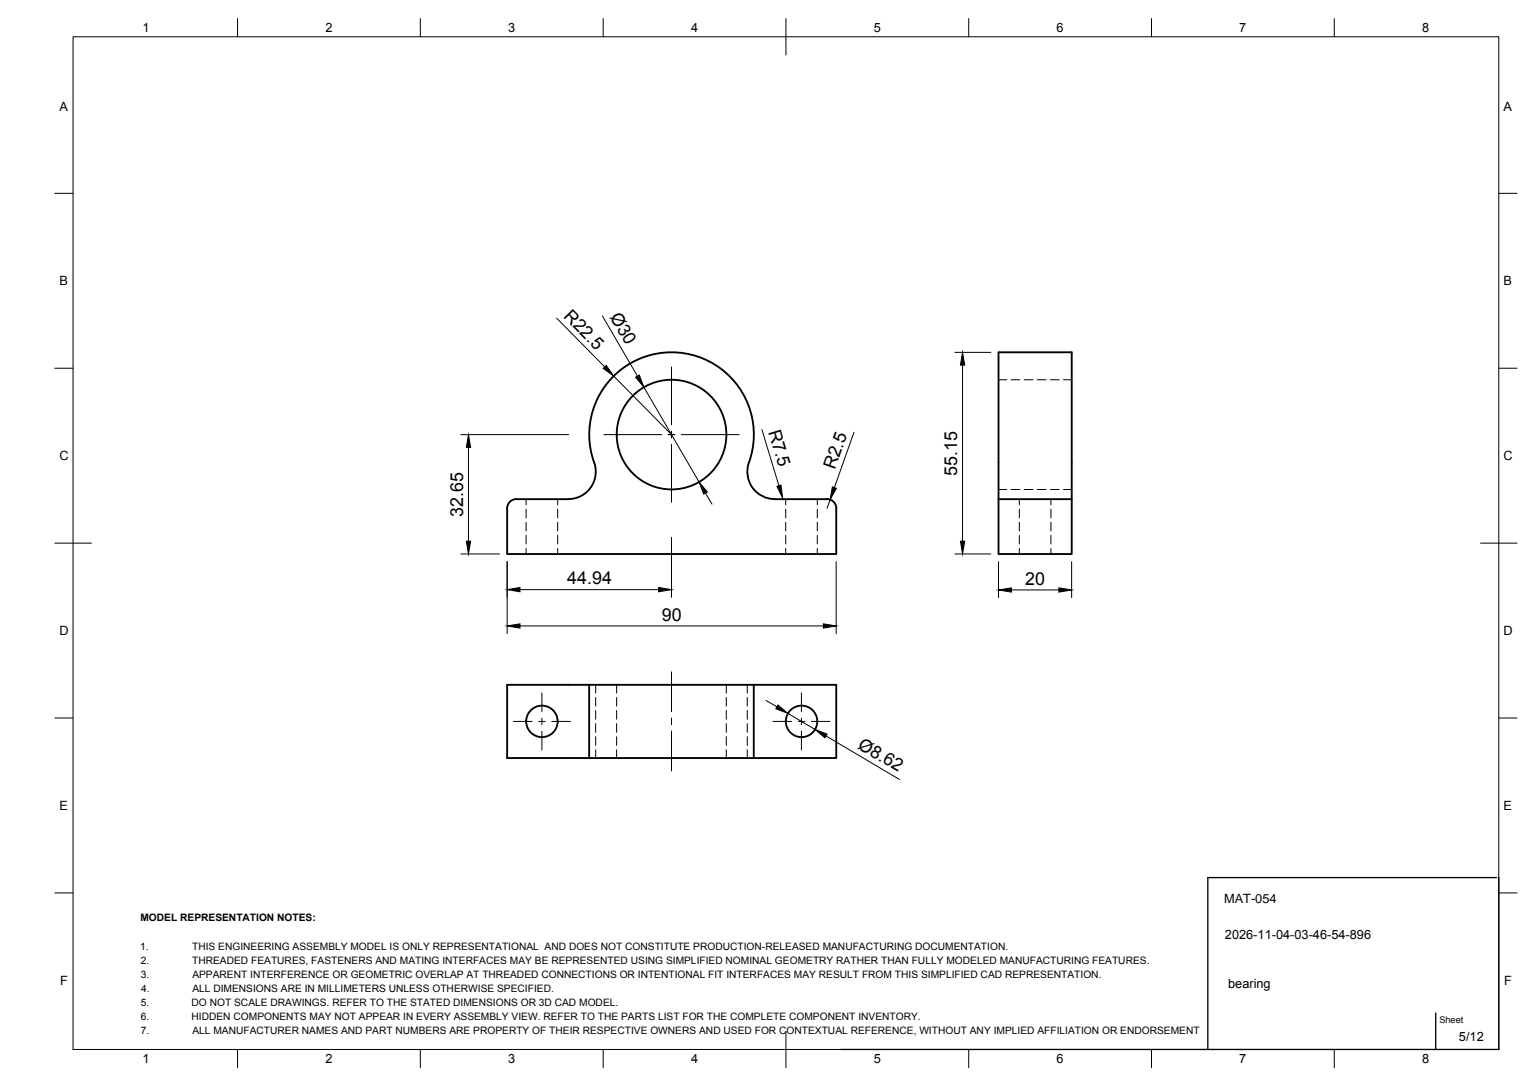
ISO-10303-21;
HEADER;
FILE_DESCRIPTION (('STEP AP214'),
    '1' );
FILE_NAME ('bearing.step',
    '2026-10-21T17:50:41',
    ( '' ),
    ( '' ),
    'SwSTEP 2.0',
    'SolidWorks 2026',
    '' );
FILE_SCHEMA (( 'AUTOMOTIVE_DESIGN' ));
ENDSEC;

DATA;
#98=CYLINDRICAL_SURFACE ( 'NONE', #29121, 7.500000000000000000 ) ;
#144=EDGE_LOOP ( 'NONE', ( #280, #13285, #21736, #21392, #14585, #6579, #11215, #29408, #31879, #667, #8768, #28527, #21247 ) ) ;
#179=DIRECTION ( 'NONE',  ( -0.000000000000000000, -1.000000000000000000, -0.000000000000000000 ) ) ;
#193=DIRECTION ( 'NONE',  ( 0.000000000000000000, -1.000000000000000000, 0.000000000000000000 ) ) ;
#280=ORIENTED_EDGE ( 'NONE', *, *, #30246, .T. ) ;
#297=LINE ( 'NONE', #7943, #15401 ) ;
#335=CARTESIAN_POINT ( 'NONE',  ( 0.000000000000000000, 0.000000000000000000, 0.000000000000000000 ) ) ;
#428=VECTOR ( 'NONE', #33661, 1000.000000000000000 ) ;
#588=ORIENTED_EDGE ( 'NONE', *, *, #13917, .F. ) ;
#650=VECTOR ( 'NONE', #5944, 1000.000000000000000 ) ;
#667=ORIENTED_EDGE ( 'NONE', *, *, #12403, .T. ) ;
#673=AXIS2_PLACEMENT_3D ( 'NONE', #16710, #32352, #5290 ) ;
#720=CIRCLE ( 'NONE', #7507, 7.500000000000000000 ) ;
#754=DIRECTION ( 'NONE',  ( 0.000000000000000000, 0.000000000000000000, 1.000000000000000000 ) ) ;
#776=DIRECTION ( 'NONE',  ( 0.000000000000000000, -1.000000000000000000, 0.000000000000000000 ) ) ;
#987=AXIS2_PLACEMENT_3D ( 'NONE', #7647, #179, #11034 ) ;
#1067=LINE ( 'NONE', #27933, #15226 ) ;
#1089=ORIENTED_EDGE ( 'NONE', *, *, #19291, .F. ) ;
#1148=DIRECTION ( 'NONE',  ( 1.000000000000000000, 0.000000000000000000, 0.000000000000000000 ) ) ;
#1179=FACE_BOUND ( 'NONE', #11958, .T. ) ;
#1196=DIRECTION ( 'NONE',  ( 0.000000000000000000, -1.000000000000000000, 0.000000000000000000 ) ) ;
#1238=CARTESIAN_POINT ( 'NONE',  ( 20.73027531293552528, -10.15143121711728469, 0.000000000000000000 ) ) ;
#1246=VERTEX_POINT ( 'NONE', #33189 ) ;
#1310=DIRECTION ( 'NONE',  ( 1.000000000000000000, 0.000000000000000000, -0.000000000000000000 ) ) ;
#1315=VERTEX_POINT ( 'NONE', #22523 ) ;
#1337=VERTEX_POINT ( 'NONE', #20892 ) ;
#1417=CARTESIAN_POINT ( 'NONE',  ( -35.55956070192387841, -32.65143121711728469, 14.30932821646982411 ) ) ;
#1464=ORIENTED_EDGE ( 'NONE', *, *, #2512, .T. ) ;
#1554=CIRCLE ( 'NONE', #28261, 4.309328216469825001 ) ;
#1579=DIRECTION ( 'NONE',  ( 0.000000000000000000, 0.000000000000000000, 1.000000000000000000 ) ) ;
#1590=CARTESIAN_POINT ( 'NONE',  ( 42.44043929807611448, -17.65143121711728469, 0.000000000000000000 ) ) ;
#1602=CARTESIAN_POINT ( 'NONE',  ( -45.05956070192387841, -32.65143121711728469, 20.00000000000000000 ) ) ;
#1647=EDGE_LOOP ( 'NONE', ( #35054, #12511, #7318, #1089 ) ) ;
#1650=FACE_OUTER_BOUND ( 'NONE', #15361, .T. ) ;
#1682=ORIENTED_EDGE ( 'NONE', *, *, #28659, .T. ) ;
#1703=LINE ( 'NONE', #15247, #2230 ) ;
#1786=ORIENTED_EDGE ( 'NONE', *, *, #28659, .F. ) ;
#1868=CARTESIAN_POINT ( 'NONE',  ( -42.55956070192386420, -17.65143121711728469, 0.000000000000000000 ) ) ;
#1884=FACE_OUTER_BOUND ( 'NONE', #34354, .T. ) ;
#1887=FACE_BOUND ( 'NONE', #19466, .T. ) ;
#1934=EDGE_LOOP ( 'NONE', ( #11019, #16399, #2768, #7931 ) ) ;
#1951=LINE ( 'NONE', #13005, #5578 ) ;
#2024=CIRCLE ( 'NONE', #9434, 7.500000000000000000 ) ;
#2056=VECTOR ( 'NONE', #12798, 1000.000000000000000 ) ;
#2062=ORIENTED_EDGE ( 'NONE', *, *, #16987, .T. ) ;
#2158=ADVANCED_FACE ( 'NONE', ( #26680 ), #13166, .F. ) ;
#2194=DIRECTION ( 'NONE',  ( -1.000000000000000000, 0.000000000000000000, 0.000000000000000000 ) ) ;
#2200=DIRECTION ( 'NONE',  ( 0.000000000000000000, 0.000000000000000000, 1.000000000000000000 ) ) ;
#2230=VECTOR ( 'NONE', #34272, 1000.000000000000000 ) ;
#2289=ORIENTED_EDGE ( 'NONE', *, *, #33790, .T. ) ;
#2360=AXIS2_PLACEMENT_3D ( 'NONE', #13291, #2588, #10616 ) ;
#2374=ORIENTED_EDGE ( 'NONE', *, *, #13917, .T. ) ;
#2424=ORIENTED_EDGE ( 'NONE', *, *, #14612, .T. ) ;
#2505=CIRCLE ( 'NONE', #31479, 15.00000000000000000 ) ;
#2512=EDGE_CURVE ( 'NONE', #15960, #1246, #1554, .T. ) ;
#2588=DIRECTION ( 'NONE',  ( -0.000000000000000000, -0.000000000000000000, -1.000000000000000000 ) ) ;
#2665=FACE_OUTER_BOUND ( 'NONE', #32945, .T. ) ;
#2768=ORIENTED_EDGE ( 'NONE', *, *, #19291, .T. ) ;
#2784=CARTESIAN_POINT ( 'NONE',  ( 42.44043929807611448, -20.15143121711728469, 20.00000000000000000 ) ) ;
#2906=FACE_OUTER_BOUND ( 'NONE', #15377, .T. ) ;
#3005=ORIENTED_EDGE ( 'NONE', *, *, #26043, .F. ) ;
#3145=DIRECTION ( 'NONE',  ( -0.000000000000000000, -0.000000000000000000, -1.000000000000000000 ) ) ;
#3170=DIRECTION ( 'NONE',  ( 0.000000000000000000, 0.000000000000000000, -1.000000000000000000 ) ) ;
#3183=ORIENTED_EDGE ( 'NONE', *, *, #29865, .T. ) ;
#3190=VECTOR ( 'NONE', #5924, 1000.000000000000000 ) ;
#3214=SHAPE_DEFINITION_REPRESENTATION ( #3232, #11185 ) ;
#3232=PRODUCT_DEFINITION_SHAPE ( 'NONE', 'NONE',  #30332 ) ;
#3267=DIRECTION ( 'NONE',  ( -0.000000000000000000, -0.000000000000000000, -1.000000000000000000 ) ) ;
#3274=LINE ( 'NONE', #11658, #4499 ) ;
#3536=DIRECTION ( 'NONE',  ( 1.000000000000000000, 0.000000000000000000, 0.000000000000000000 ) ) ;
#3537=ORIENTED_EDGE ( 'NONE', *, *, #17476, .T. ) ;
#3726=EDGE_CURVE ( 'NONE', #14044, #25632, #1951, .T. ) ;
#3731=VECTOR ( 'NONE', #32637, 1000.000000000000000 ) ;
#3774=CIRCLE ( 'NONE', #26508, 4.309328216469825001 ) ;
#3834=CIRCLE ( 'NONE', #33395, 4.309328216469825001 ) ;
#4017=FACE_BOUND ( 'NONE', #34001, .T. ) ;
#4073=CIRCLE ( 'NONE', #6902, 7.500000000000000000 ) ;
#4099=CARTESIAN_POINT ( 'NONE',  ( -42.55956070192386420, -17.65143121711728469, 20.00000000000000000 ) ) ;
#4161=CARTESIAN_POINT ( 'NONE',  ( 0.000000000000000000, 0.000000000000000000, 20.00000000000000000 ) ) ;
#4275=CARTESIAN_POINT ( 'NONE',  ( 0.000000000000000000, 0.000000000000000000, 20.00000000000000000 ) ) ;
#4282=DIRECTION ( 'NONE',  ( 0.000000000000000000, 0.000000000000000000, 1.000000000000000000 ) ) ;
#4476=CYLINDRICAL_SURFACE ( 'NONE', #23230, 7.500000000000000000 ) ;
#4482=DIRECTION ( 'NONE',  ( 0.000000000000000000, 1.000000000000000000, 0.000000000000000000 ) ) ;
#4499=VECTOR ( 'NONE', #5934, 1000.000000000000000 ) ;
#4571=VERTEX_POINT ( 'NONE', #32067 ) ;
#4572=CARTESIAN_POINT ( 'NONE',  ( -42.55956070192386420, -17.65143121711728469, 0.000000000000000000 ) ) ;
#4576=FACE_OUTER_BOUND ( 'NONE', #1934, .T. ) ;
#4606=VERTEX_POINT ( 'NONE', #26730 ) ;
#4611=DIRECTION ( 'NONE',  ( 0.000000000000000000, 0.000000000000000000, 1.000000000000000000 ) ) ;
#4856=CARTESIAN_POINT ( 'NONE',  ( -28.23027531293552528, -10.15143121711728469, 20.00000000000000000 ) ) ;
#4884=AXIS2_PLACEMENT_3D ( 'NONE', #10644, #13141, #23974 ) ;
#4893=EDGE_LOOP ( 'NONE', ( #17206, #26632 ) ) ;
#4899=DIRECTION ( 'NONE',  ( -0.000000000000000000, -0.000000000000000000, -1.000000000000000000 ) ) ;
#4963=ORIENTED_EDGE ( 'NONE', *, *, #20775, .T. ) ;
#5064=CARTESIAN_POINT ( 'NONE',  ( 44.94043929807611448, -32.65143121711728469, 20.00000000000000000 ) ) ;
#5074=CYLINDRICAL_SURFACE ( 'NONE', #6927, 4.309328216469825001 ) ;
#5186=DIRECTION ( 'NONE',  ( -0.000000000000000000, -1.000000000000000000, -0.000000000000000000 ) ) ;
#5189=EDGE_CURVE ( 'NONE', #20760, #34690, #26627, .T. ) ;
#5290=DIRECTION ( 'NONE',  ( 1.000000000000000000, 0.000000000000000000, 0.000000000000000000 ) ) ;
#5355=EDGE_LOOP ( 'NONE', ( #4963, #33386, #10408, #3537 ) ) ;
#5426=DIRECTION ( 'NONE',  ( -1.000000000000000000, 0.000000000000000000, 0.000000000000000000 ) ) ;
#5445=ORIENTED_EDGE ( 'NONE', *, *, #19569, .F. ) ;
#5578=VECTOR ( 'NONE', #23841, 1000.000000000000000 ) ;
#5591=CYLINDRICAL_SURFACE ( 'NONE', #25040, 4.309328216469825001 ) ;
#5624=EDGE_CURVE ( 'NONE', #17462, #1337, #3834, .T. ) ;
#5658=LINE ( 'NONE', #32062, #17725 ) ;
#5665=DIRECTION ( 'NONE',  ( 1.000000000000000000, 0.000000000000000000, 0.000000000000000000 ) ) ;
#5735=CIRCLE ( 'NONE', #12609, 7.500000000000000000 ) ;
#5746=AXIS2_PLACEMENT_3D ( 'NONE', #13699, #29902, #5665 ) ;
#5924=DIRECTION ( 'NONE',  ( -0.000000000000000000, -0.000000000000000000, -1.000000000000000000 ) ) ;
#5934=DIRECTION ( 'NONE',  ( 1.000000000000000000, 0.000000000000000000, 0.000000000000000000 ) ) ;
#5944=DIRECTION ( 'NONE',  ( -0.000000000000000000, -0.000000000000000000, -1.000000000000000000 ) ) ;
#5953=VECTOR ( 'NONE', #24547, 1000.000000000000000 ) ;
#5995=ORIENTED_EDGE ( 'NONE', *, *, #7093, .F. ) ;
#6095=VECTOR ( 'NONE', #4482, 1000.000000000000000 ) ;
#6135=ORIENTED_EDGE ( 'NONE', *, *, #30246, .F. ) ;
#6166=EDGE_CURVE ( 'NONE', #30767, #27908, #24708, .T. ) ;
#6275=DIRECTION ( 'NONE',  ( -1.000000000000000000, 0.000000000000000000, 0.000000000000000000 ) ) ;
#6422=ORIENTED_EDGE ( 'NONE', *, *, #5189, .T. ) ;
#6476=DIRECTION ( 'NONE',  ( 0.000000000000000000, 0.000000000000000000, -1.000000000000000000 ) ) ;
#6579=ORIENTED_EDGE ( 'NONE', *, *, #35041, .T. ) ;
#6732=AXIS2_PLACEMENT_3D ( 'NONE', #11381, #11213, #30241 ) ;
#6779=LINE ( 'NONE', #31683, #25200 ) ;
#6823=DIRECTION ( 'NONE',  ( 0.000000000000000000, 0.000000000000000000, 1.000000000000000000 ) ) ;
#6879=AXIS2_PLACEMENT_3D ( 'NONE', #14649, #22815, #9288 ) ;
#6902=AXIS2_PLACEMENT_3D ( 'NONE', #14201, #3145, #22373 ) ;
#6904=ADVANCED_FACE ( 'NONE', ( #17929, #1179, #20062 ), #28755, .F. ) ;
#6907=ORIENTED_EDGE ( 'NONE', *, *, #26043, .T. ) ;
#6926=CARTESIAN_POINT ( 'NONE',  ( 44.94043929807611448, -20.15143121711728469, 20.00000000000000000 ) ) ;
#6927=AXIS2_PLACEMENT_3D ( 'NONE', #15795, #26623, #10431 ) ;
#6956=PLANE ( 'NONE',  #7053 ) ;
#7022=DIRECTION ( 'NONE',  ( 0.000000000000000000, -1.000000000000000000, 0.000000000000000000 ) ) ;
#7048=ORIENTED_EDGE ( 'NONE', *, *, #7445, .F. ) ;
#7053=AXIS2_PLACEMENT_3D ( 'NONE', #17847, #28681, #4282 ) ;
#7057=ORIENTED_EDGE ( 'NONE', *, *, #10691, .T. ) ;
#7075=LINE ( 'NONE', #9239, #10341 ) ;
#7093=EDGE_CURVE ( 'NONE', #11385, #31447, #18617, .T. ) ;
#7134=ORIENTED_EDGE ( 'NONE', *, *, #31070, .T. ) ;
#7156=CYLINDRICAL_SURFACE ( 'NONE', #27609, 2.500000000000002220 ) ;
#7177=DIRECTION ( 'NONE',  ( -1.000000000000000000, 0.000000000000000000, 0.000000000000000000 ) ) ;
#7238=EDGE_CURVE ( 'NONE', #29888, #25980, #21788, .T. ) ;
#7318=ORIENTED_EDGE ( 'NONE', *, *, #16987, .F. ) ;
#7422=CARTESIAN_POINT ( 'NONE',  ( -35.55956070192387841, -32.65143121711728469, 5.690671783530174999 ) ) ;
#7443=ADVANCED_FACE ( 'NONE', ( #29590 ), #7156, .T. ) ;
#7444=CARTESIAN_POINT ( 'NONE',  ( 20.73027531293552528, -10.15143121711728469, 20.00000000000000000 ) ) ;
#7445=EDGE_CURVE ( 'NONE', #1337, #23936, #18061, .T. ) ;
#7470=CARTESIAN_POINT ( 'NONE',  ( 28.23027531293552528, -17.65143121711728469, 20.00000000000000000 ) ) ;
#7507=AXIS2_PLACEMENT_3D ( 'NONE', #4856, #33412, #17247 ) ;
#7509=DIRECTION ( 'NONE',  ( -0.000000000000000000, -0.000000000000000000, -1.000000000000000000 ) ) ;
#7524=VERTEX_POINT ( 'NONE', #31724 ) ;
#7588=CARTESIAN_POINT ( 'NONE',  ( -28.23027531293552528, -17.65143121711728469, 0.000000000000000000 ) ) ;
#7601=ORIENTED_EDGE ( 'NONE', *, *, #32770, .T. ) ;
#7647=CARTESIAN_POINT ( 'NONE',  ( -35.55956070192387841, -12.65143121711728291, 10.00000000000000000 ) ) ;
#7706=FACE_OUTER_BOUND ( 'NONE', #21398, .T. ) ;
#7751=FACE_OUTER_BOUND ( 'NONE', #24508, .T. ) ;
#7754=EDGE_CURVE ( 'NONE', #25273, #4606, #23458, .T. ) ;
#7759=VERTEX_POINT ( 'NONE', #7422 ) ;
#7760=CARTESIAN_POINT ( 'NONE',  ( 44.94043929807611448, -32.65143121711728469, 20.00000000000000000 ) ) ;
#7854=EDGE_CURVE ( 'NONE', #1246, #15960, #21952, .T. ) ;
#7931=ORIENTED_EDGE ( 'NONE', *, *, #32770, .F. ) ;
#7943=CARTESIAN_POINT ( 'NONE',  ( -28.23027531293552528, -17.65143121711728469, 20.00000000000000000 ) ) ;
#7968=DIRECTION ( 'NONE',  ( -0.000000000000000000, -0.000000000000000000, -1.000000000000000000 ) ) ;
#8026=CIRCLE ( 'NONE', #22831, 22.50000000000000355 ) ;
#8101=EDGE_CURVE ( 'NONE', #23708, #12488, #31623, .T. ) ;
#8204=( LENGTH_UNIT ( ) NAMED_UNIT ( * ) SI_UNIT ( .MILLI., .METRE. ) );
#8240=ORIENTED_EDGE ( 'NONE', *, *, #27319, .F. ) ;
#8255=FACE_OUTER_BOUND ( 'NONE', #9278, .T. ) ;
#8459=CIRCLE ( 'NONE', #32889, 15.00000000000000000 ) ;
#8477=ORIENTED_EDGE ( 'NONE', *, *, #9298, .F. ) ;
#8589=ORIENTED_EDGE ( 'NONE', *, *, #15548, .F. ) ;
#8658=DIRECTION ( 'NONE',  ( 0.000000000000000000, 0.000000000000000000, 1.000000000000000000 ) ) ;
#8665=AXIS2_PLACEMENT_3D ( 'NONE', #21239, #27510, #2194 ) ;
#8673=CARTESIAN_POINT ( 'NONE',  ( -45.05956070192387841, -20.15143121711730245, 0.000000000000000000 ) ) ;
#8704=EDGE_CURVE ( 'NONE', #27908, #4571, #12193, .T. ) ;
#8709=DIRECTION ( 'NONE',  ( 0.000000000000000000, 0.000000000000000000, -1.000000000000000000 ) ) ;
#8768=ORIENTED_EDGE ( 'NONE', *, *, #7754, .T. ) ;
#8858=VECTOR ( 'NONE', #28004, 1000.000000000000000 ) ;
#9037=STYLED_ITEM('',(#35275),#10712);
#9038=EDGE_CURVE ( 'NONE', #26426, #14044, #15163, .T. ) ;
#9046=DIRECTION ( 'NONE',  ( -0.000000000000000000, -1.000000000000000000, -0.000000000000000000 ) ) ;
#9063=DIRECTION ( 'NONE',  ( -1.000000000000000000, -0.000000000000000000, -0.000000000000000000 ) ) ;
#9153=AXIS2_PLACEMENT_3D ( 'NONE', #12764, #9563, #18280 ) ;
#9239=CARTESIAN_POINT ( 'NONE',  ( -42.55956070192386420, -17.65143121711728469, 20.00000000000000000 ) ) ;
#9278=EDGE_LOOP ( 'NONE', ( #3183, #24989, #30938, #30551 ) ) ;
#9288=DIRECTION ( 'NONE',  ( -1.000000000000000000, 0.000000000000000000, 0.000000000000000000 ) ) ;
#9298=EDGE_CURVE ( 'NONE', #25980, #7524, #24542, .T. ) ;
#9371=AXIS2_PLACEMENT_3D ( 'NONE', #23997, #9046, #3170 ) ;
#9421=CARTESIAN_POINT ( 'NONE',  ( -45.05956070192387841, -32.65143121711728469, 20.00000000000000000 ) ) ;
#9434=AXIS2_PLACEMENT_3D ( 'NONE', #10634, #15983, #18825 ) ;
#9505=CARTESIAN_POINT ( 'NONE',  ( 44.94043929807611448, -20.15143121711728469, 0.000000000000000000 ) ) ;
#9535=EDGE_CURVE ( 'NONE', #33194, #31447, #1067, .T. ) ;
#9563=DIRECTION ( 'NONE',  ( -0.000000000000000000, 0.000000000000000000, -1.000000000000000000 ) ) ;
#9610=CARTESIAN_POINT ( 'NONE',  ( -45.05956070192387841, -20.15143121711730245, 0.000000000000000000 ) ) ;
#9779=ORIENTED_EDGE ( 'NONE', *, *, #29342, .T. ) ;
#9841=LINE ( 'NONE', #23542, #6095 ) ;
#9842=CARTESIAN_POINT ( 'NONE',  ( -42.55956070192387841, -20.15143121711728469, 20.00000000000000000 ) ) ;
#9855=CYLINDRICAL_SURFACE ( 'NONE', #8665, 22.50000000000000355 ) ;
#9862=DIRECTION ( 'NONE',  ( 0.000000000000000000, -1.000000000000000000, 0.000000000000000000 ) ) ;
#9884=PRODUCT_DEFINITION_FORMATION_WITH_SPECIFIED_SOURCE ( 'ANY', '', #16613, .NOT_KNOWN. ) ;
#9992=VERTEX_POINT ( 'NONE', #7444 ) ;
#10012=CARTESIAN_POINT ( 'NONE',  ( -35.55956070192387841, -32.65143121711728469, 10.00000000000000000 ) ) ;
#10085=ORIENTED_EDGE ( 'NONE', *, *, #5624, .F. ) ;
#10100=FACE_OUTER_BOUND ( 'NONE', #1647, .T. ) ;
#10195=CARTESIAN_POINT ( 'NONE',  ( 42.44043929807611448, -17.65143121711728469, 20.00000000000000000 ) ) ;
#10202=CARTESIAN_POINT ( 'NONE',  ( -45.05956070192387841, -32.65143121711728469, 0.000000000000000000 ) ) ;
#10261=ORIENTED_EDGE ( 'NONE', *, *, #24371, .F. ) ;
#10271=DIRECTION ( 'NONE',  ( -1.000000000000000000, 0.000000000000000000, 0.000000000000000000 ) ) ;
#10293=CARTESIAN_POINT ( 'NONE',  ( 0.000000000000000000, 0.000000000000000000, 20.00000000000000000 ) ) ;
#10341=VECTOR ( 'NONE', #9063, 1000.000000000000000 ) ;
#10358=EDGE_LOOP ( 'NONE', ( #28928, #26404, #12720, #20054 ) ) ;
#10408=ORIENTED_EDGE ( 'NONE', *, *, #7754, .F. ) ;
#10431=DIRECTION ( 'NONE',  ( 0.000000000000000000, 0.000000000000000000, -1.000000000000000000 ) ) ;
#10543=( NAMED_UNIT ( * ) PLANE_ANGLE_UNIT ( ) SI_UNIT ( $, .RADIAN. ) );
#10581=EDGE_LOOP ( 'NONE', ( #8589, #12296, #11638, #8240 ) ) ;
#10616=DIRECTION ( 'NONE',  ( -1.000000000000000000, 0.000000000000000000, 0.000000000000000000 ) ) ;
#10634=CARTESIAN_POINT ( 'NONE',  ( 28.23027531293552528, -10.15143121711728469, 0.000000000000000000 ) ) ;
#10644=CARTESIAN_POINT ( 'NONE',  ( 35.44043929807611448, -17.65143121711728469, 10.00000000000000000 ) ) ;
#10669=DIRECTION ( 'NONE',  ( 0.000000000000000000, 0.000000000000000000, 1.000000000000000000 ) ) ;
#10677=ORIENTED_EDGE ( 'NONE', *, *, #9535, .F. ) ;
#10691=EDGE_CURVE ( 'NONE', #16381, #1315, #15322, .T. ) ;
#10712=MANIFOLD_SOLID_BREP ( 'Cut-Extrude1', #29869 ) ;
#10929=( GEOMETRIC_REPRESENTATION_CONTEXT ( 3 ) GLOBAL_UNCERTAINTY_ASSIGNED_CONTEXT ( ( #28468 ) ) GLOBAL_UNIT_ASSIGNED_CONTEXT ( ( #14663, #30490, #31015 ) ) REPRESENTATION_CONTEXT ( 'NONE', 'WORKASPACE' ) );
#11019=ORIENTED_EDGE ( 'NONE', *, *, #8704, .F. ) ;
#11034=DIRECTION ( 'NONE',  ( 0.000000000000000000, 0.000000000000000000, -1.000000000000000000 ) ) ;
#11068=( NAMED_UNIT ( * ) SI_UNIT ( $, .STERADIAN. ) SOLID_ANGLE_UNIT ( ) );
#11140=LINE ( 'NONE', #33538, #650 ) ;
#11171=ORIENTED_EDGE ( 'NONE', *, *, #7093, .T. ) ;
#11185=SHAPE_REPRESENTATION ( 'bearing', ( #28566 ), #10929 ) ;
#11213=DIRECTION ( 'NONE',  ( 0.000000000000000000, 0.000000000000000000, 1.000000000000000000 ) ) ;
#11215=ORIENTED_EDGE ( 'NONE', *, *, #30006, .T. ) ;
#11232=DIRECTION ( 'NONE',  ( 0.000000000000000000, 0.000000000000000000, -1.000000000000000000 ) ) ;
#11298=CARTESIAN_POINT ( 'NONE',  ( 28.23027531293552528, -17.65143121711728469, 20.00000000000000000 ) ) ;
#11330=ADVANCED_FACE ( 'NONE', ( #10100 ), #18307, .F. ) ;
#11332=( GEOMETRIC_REPRESENTATION_CONTEXT ( 3 ) GLOBAL_UNCERTAINTY_ASSIGNED_CONTEXT ( ( #31933 ) ) GLOBAL_UNIT_ASSIGNED_CONTEXT ( ( #8204, #10543, #11068 ) ) REPRESENTATION_CONTEXT ( 'NONE', 'WORKASPACE' ) );
#11381=CARTESIAN_POINT ( 'NONE',  ( 42.44043929807611448, -20.15143121711728469, 0.000000000000000000 ) ) ;
#11385=VERTEX_POINT ( 'NONE', #7588 ) ;
#11495=AXIS2_PLACEMENT_3D ( 'NONE', #30693, #24981, #1148 ) ;
#11619=FACE_OUTER_BOUND ( 'NONE', #144, .T. ) ;
#11636=EDGE_LOOP ( 'NONE', ( #29071, #13902, #19431, #7057 ) ) ;
#11638=ORIENTED_EDGE ( 'NONE', *, *, #18730, .T. ) ;
#11658=CARTESIAN_POINT ( 'NONE',  ( -45.05956070192387841, -32.65143121711728469, 0.000000000000000000 ) ) ;
#11690=ORIENTED_EDGE ( 'NONE', *, *, #15800, .F. ) ;
#11754=DIRECTION ( 'NONE',  ( 0.000000000000000000, -1.000000000000000000, 0.000000000000000000 ) ) ;
#11833=LINE ( 'NONE', #16643, #8858 ) ;
#11844=CARTESIAN_POINT ( 'NONE',  ( 15.00000000000000000, 1.836970198721029589E-15, 20.00000000000000000 ) ) ;
#11955=VECTOR ( 'NONE', #32052, 1000.000000000000000 ) ;
#11958=EDGE_LOOP ( 'NONE', ( #1786, #32913 ) ) ;
#11980=ADVANCED_FACE ( 'NONE', ( #2906 ), #27653, .T. ) ;
#12006=CIRCLE ( 'NONE', #17143, 4.309328216469825001 ) ;
#12034=ADVANCED_FACE ( 'NONE', ( #25862 ), #33695, .F. ) ;
#12058=ADVANCED_FACE ( 'NONE', ( #1650 ), #4476, .F. ) ;
#12193=LINE ( 'NONE', #11844, #13398 ) ;
#12248=PLANE ( 'NONE',  #9153 ) ;
#12252=CARTESIAN_POINT ( 'NONE',  ( -42.55956070192386420, -17.65143121711728469, 20.00000000000000000 ) ) ;
#12296=ORIENTED_EDGE ( 'NONE', *, *, #13818, .T. ) ;
#12403=EDGE_CURVE ( 'NONE', #14044, #25273, #30948, .T. ) ;
#12449=CARTESIAN_POINT ( 'NONE',  ( -21.17270648470164218, -7.613573412837966181, 20.00000000000000000 ) ) ;
#12488=VERTEX_POINT ( 'NONE', #12449 ) ;
#12491=DIRECTION ( 'NONE',  ( 1.000000000000000000, 0.000000000000000000, 0.000000000000000000 ) ) ;
#12511=ORIENTED_EDGE ( 'NONE', *, *, #8704, .T. ) ;
#12519=CARTESIAN_POINT ( 'NONE',  ( 28.23027531293552528, -10.15143121711728469, 20.00000000000000000 ) ) ;
#12564=DIRECTION ( 'NONE',  ( 0.000000000000000000, 0.000000000000000000, 1.000000000000000000 ) ) ;
#12609=AXIS2_PLACEMENT_3D ( 'NONE', #34128, #20273, #17448 ) ;
#12720=ORIENTED_EDGE ( 'NONE', *, *, #30005, .F. ) ;
#12764=CARTESIAN_POINT ( 'NONE',  ( 28.23027531293552528, -10.15143121711728469, 0.000000000000000000 ) ) ;
#12768=FACE_OUTER_BOUND ( 'NONE', #15181, .T. ) ;
#12798=DIRECTION ( 'NONE',  ( 0.000000000000000000, 1.000000000000000000, 0.000000000000000000 ) ) ;
#12799=EDGE_CURVE ( 'NONE', #27908, #30767, #8459, .T. ) ;
#12846=DIRECTION ( 'NONE',  ( -0.000000000000000000, -1.000000000000000000, -0.000000000000000000 ) ) ;
#12907=EDGE_CURVE ( 'NONE', #12488, #32903, #1703, .T. ) ;
#13005=CARTESIAN_POINT ( 'NONE',  ( -45.05956070192387841, -32.65143121711728469, 20.00000000000000000 ) ) ;
#13052=DIRECTION ( 'NONE',  ( -0.000000000000000000, -0.000000000000000000, -1.000000000000000000 ) ) ;
#13073=DIRECTION ( 'NONE',  ( 1.000000000000000000, 0.000000000000000000, 0.000000000000000000 ) ) ;
#13093=VECTOR ( 'NONE', #21913, 1000.000000000000000 ) ;
#13141=DIRECTION ( 'NONE',  ( 0.000000000000000000, -1.000000000000000000, 0.000000000000000000 ) ) ;
#13144=EDGE_CURVE ( 'NONE', #25632, #15499, #3274, .T. ) ;
#13166=CYLINDRICAL_SURFACE ( 'NONE', #9371, 4.309328216469825001 ) ;
#13205=FACE_OUTER_BOUND ( 'NONE', #11636, .T. ) ;
#13212=CARTESIAN_POINT ( 'NONE',  ( 20.73027531293552528, -10.15143121711728469, 20.00000000000000000 ) ) ;
#13219=DIRECTION ( 'NONE',  ( 0.000000000000000000, 0.000000000000000000, -1.000000000000000000 ) ) ;
#13250=AXIS2_PLACEMENT_3D ( 'NONE', #22071, #11754, #8709 ) ;
#13285=ORIENTED_EDGE ( 'NONE', *, *, #15548, .T. ) ;
#13291=CARTESIAN_POINT ( 'NONE',  ( 42.44043929807611448, -20.15143121711728469, 20.00000000000000000 ) ) ;
#13398=VECTOR ( 'NONE', #33529, 1000.000000000000000 ) ;
#13457=FACE_OUTER_BOUND ( 'NONE', #28066, .T. ) ;
#13479=DIRECTION ( 'NONE',  ( -1.000000000000000000, 0.000000000000000000, 0.000000000000000000 ) ) ;
#13697=ORIENTED_EDGE ( 'NONE', *, *, #8101, .F. ) ;
#13699=CARTESIAN_POINT ( 'NONE',  ( -28.23027531293552528, -10.15143121711728469, 0.000000000000000000 ) ) ;
#13700=VERTEX_POINT ( 'NONE', #14834 ) ;
#13818=EDGE_CURVE ( 'NONE', #9992, #23016, #29221, .T. ) ;
#13851=ORIENTED_EDGE ( 'NONE', *, *, #5189, .F. ) ;
#13902=ORIENTED_EDGE ( 'NONE', *, *, #22751, .F. ) ;
#13917=EDGE_CURVE ( 'NONE', #17462, #7759, #27774, .T. ) ;
#14026=EDGE_CURVE ( 'NONE', #4606, #20760, #22968, .T. ) ;
#14036=DIRECTION ( 'NONE',  ( 1.000000000000000000, 0.000000000000000000, 0.000000000000000000 ) ) ;
#14044=VERTEX_POINT ( 'NONE', #1602 ) ;
#14102=VERTEX_POINT ( 'NONE', #28313 ) ;
#14201=CARTESIAN_POINT ( 'NONE',  ( 28.23027531293552528, -10.15143121711728469, 20.00000000000000000 ) ) ;
#14349=AXIS2_PLACEMENT_3D ( 'NONE', #2784, #18828, #13479 ) ;
#14500=DIRECTION ( 'NONE',  ( -1.000000000000000000, 0.000000000000000000, 0.000000000000000000 ) ) ;
#14585=ORIENTED_EDGE ( 'NONE', *, *, #8101, .T. ) ;
#14612=EDGE_CURVE ( 'NONE', #18684, #11385, #297, .T. ) ;
#14649=CARTESIAN_POINT ( 'NONE',  ( 28.23027531293552528, -10.15143121711728469, 20.00000000000000000 ) ) ;
#14663=( LENGTH_UNIT ( ) NAMED_UNIT ( * ) SI_UNIT ( .MILLI., .METRE. ) );
#14730=DIRECTION ( 'NONE',  ( 0.000000000000000000, 1.000000000000000000, 0.000000000000000000 ) ) ;
#14833=VECTOR ( 'NONE', #15910, 1000.000000000000000 ) ;
#14834=CARTESIAN_POINT ( 'NONE',  ( 22.50000000000000355, 2.755455298081545172E-15, 20.00000000000000000 ) ) ;
#14862=CARTESIAN_POINT ( 'NONE',  ( -15.00000000000000000, 0.000000000000000000, 20.00000000000000000 ) ) ;
#14946=EDGE_LOOP ( 'NONE', ( #34225, #32974, #6907, #1682 ) ) ;
#15050=DIRECTION ( 'NONE',  ( -0.000000000000000000, -0.000000000000000000, -1.000000000000000000 ) ) ;
#15068=CARTESIAN_POINT ( 'NONE',  ( -35.55956070192387841, -17.65143121711728469, 10.00000000000000000 ) ) ;
#15080=EDGE_CURVE ( 'NONE', #1337, #17462, #12006, .T. ) ;
#15127=CARTESIAN_POINT ( 'NONE',  ( -45.05956070192387841, -20.15143121711730245, 20.00000000000000000 ) ) ;
#15163=LINE ( 'NONE', #27972, #428 ) ;
#15181=EDGE_LOOP ( 'NONE', ( #11171, #10677, #27068, #2424 ) ) ;
#15226=VECTOR ( 'NONE', #22776, 1000.000000000000000 ) ;
#15244=ORIENTED_EDGE ( 'NONE', *, *, #29080, .F. ) ;
#15245=CARTESIAN_POINT ( 'NONE',  ( -45.05956070192387841, -32.65143121711728469, 20.00000000000000000 ) ) ;
#15247=CARTESIAN_POINT ( 'NONE',  ( -21.17270648470164218, -7.613573412837966181, 20.00000000000000000 ) ) ;
#15258=ORIENTED_EDGE ( 'NONE', *, *, #7445, .T. ) ;
#15272=ORIENTED_EDGE ( 'NONE', *, *, #13144, .F. ) ;
#15322=CIRCLE ( 'NONE', #27223, 22.50000000000000355 ) ;
#15361=EDGE_LOOP ( 'NONE', ( #31637, #6135, #15564, #24418 ) ) ;
#15377=EDGE_LOOP ( 'NONE', ( #22640, #17518, #27219, #21030 ) ) ;
#15401=VECTOR ( 'NONE', #24473, 1000.000000000000000 ) ;
#15404=EDGE_CURVE ( 'NONE', #34690, #7524, #5658, .T. ) ;
#15499=VERTEX_POINT ( 'NONE', #28276 ) ;
#15548=EDGE_CURVE ( 'NONE', #9992, #27517, #5735, .T. ) ;
#15563=CIRCLE ( 'NONE', #19555, 4.309328216469825001 ) ;
#15564=ORIENTED_EDGE ( 'NONE', *, *, #9298, .T. ) ;
#15610=VERTEX_POINT ( 'NONE', #23122 ) ;
#15612=PLANE ( 'NONE',  #23405 ) ;
#15640=ORIENTED_EDGE ( 'NONE', *, *, #7854, .T. ) ;
#15794=APPLICATION_CONTEXT ( 'automotive_design' ) ;
#15795=CARTESIAN_POINT ( 'NONE',  ( 35.44043929807611448, -12.65143121711728291, 10.00000000000000000 ) ) ;
#15800=EDGE_CURVE ( 'NONE', #4606, #29888, #26821, .T. ) ;
#15868=EDGE_LOOP ( 'NONE', ( #15640, #1464 ) ) ;
#15910=DIRECTION ( 'NONE',  ( -0.000000000000000000, -1.000000000000000000, -0.000000000000000000 ) ) ;
#15960=VERTEX_POINT ( 'NONE', #31250 ) ;
#15983=DIRECTION ( 'NONE',  ( -0.000000000000000000, -0.000000000000000000, -1.000000000000000000 ) ) ;
#16048=CARTESIAN_POINT ( 'NONE',  ( 21.17270648470164218, -7.613573412837960852, 20.00000000000000000 ) ) ;
#16096=EDGE_CURVE ( 'NONE', #13700, #23708, #19947, .T. ) ;
#16206=CARTESIAN_POINT ( 'NONE',  ( 0.000000000000000000, 0.000000000000000000, 20.00000000000000000 ) ) ;
#16381=VERTEX_POINT ( 'NONE', #30857 ) ;
#16399=ORIENTED_EDGE ( 'NONE', *, *, #12799, .T. ) ;
#16413=CARTESIAN_POINT ( 'NONE',  ( 35.44043929807611448, -32.65143121711728469, 10.00000000000000000 ) ) ;
#16428=DIRECTION ( 'NONE',  ( 1.000000000000000000, 0.000000000000000000, 0.000000000000000000 ) ) ;
#16552=EDGE_CURVE ( 'NONE', #29888, #34690, #26559, .T. ) ;
#16613=PRODUCT ( 'bearing', 'bearing', '', ( #32579 ) ) ;
#16643=CARTESIAN_POINT ( 'NONE',  ( -15.00000000000000000, 0.000000000000000000, 20.00000000000000000 ) ) ;
#16710=CARTESIAN_POINT ( 'NONE',  ( 0.000000000000000000, 0.000000000000000000, 0.000000000000000000 ) ) ;
#16753=LINE ( 'NONE', #16048, #5953 ) ;
#16987=EDGE_CURVE ( 'NONE', #14102, #4571, #26360, .T. ) ;
#17072=ORIENTED_EDGE ( 'NONE', *, *, #15404, .F. ) ;
#17143=AXIS2_PLACEMENT_3D ( 'NONE', #20180, #776, #30316 ) ;
#17172=CARTESIAN_POINT ( 'NONE',  ( -28.23027531293552528, -10.15143121711728469, 20.00000000000000000 ) ) ;
#17206=ORIENTED_EDGE ( 'NONE', *, *, #6166, .F. ) ;
#17247=DIRECTION ( 'NONE',  ( 1.000000000000000000, 0.000000000000000000, 0.000000000000000000 ) ) ;
#17339=EDGE_LOOP ( 'NONE', ( #27742, #8477, #27793, #30665 ) ) ;
#17344=VERTEX_POINT ( 'NONE', #20950 ) ;
#17383=AXIS2_PLACEMENT_3D ( 'NONE', #15245, #14730, #25733 ) ;
#17418=ORIENTED_EDGE ( 'NONE', *, *, #30777, .F. ) ;
#17448=DIRECTION ( 'NONE',  ( -1.000000000000000000, 0.000000000000000000, 0.000000000000000000 ) ) ;
#17462=VERTEX_POINT ( 'NONE', #29317 ) ;
#17476=EDGE_CURVE ( 'NONE', #25273, #15499, #32492, .T. ) ;
#17518=ORIENTED_EDGE ( 'NONE', *, *, #27807, .T. ) ;
#17533=DIRECTION ( 'NONE',  ( -0.000000000000000000, 0.000000000000000000, -1.000000000000000000 ) ) ;
#17572=ORIENTED_EDGE ( 'NONE', *, *, #14026, .T. ) ;
#17575=DIRECTION ( 'NONE',  ( 0.000000000000000000, 0.000000000000000000, -1.000000000000000000 ) ) ;
#17725=VECTOR ( 'NONE', #34745, 1000.000000000000000 ) ;
#17819=ORIENTED_EDGE ( 'NONE', *, *, #10691, .F. ) ;
#17846=CARTESIAN_POINT ( 'NONE',  ( -22.50000000000000355, 0.000000000000000000, 20.00000000000000000 ) ) ;
#17847=CARTESIAN_POINT ( 'NONE',  ( 44.94043929807611448, -32.65143121711728469, 20.00000000000000000 ) ) ;
#17929=FACE_BOUND ( 'NONE', #22601, .T. ) ;
#18061=LINE ( 'NONE', #23543, #32161 ) ;
#18238=CARTESIAN_POINT ( 'NONE',  ( -22.50000000000000355, 0.000000000000000000, 0.000000000000000000 ) ) ;
#18280=DIRECTION ( 'NONE',  ( -1.000000000000000000, 0.000000000000000000, 0.000000000000000000 ) ) ;
#18307=CYLINDRICAL_SURFACE ( 'NONE', #31134, 15.00000000000000000 ) ;
#18422=EDGE_LOOP ( 'NONE', ( #31903, #27595, #33467, #2289 ) ) ;
#18512=CARTESIAN_POINT ( 'NONE',  ( 22.50000000000000355, 2.755455298081545172E-15, 20.00000000000000000 ) ) ;
#18569=CARTESIAN_POINT ( 'NONE',  ( 0.000000000000000000, 0.000000000000000000, 0.000000000000000000 ) ) ;
#18617=LINE ( 'NONE', #1868, #24176 ) ;
#18654=CARTESIAN_POINT ( 'NONE',  ( -28.23027531293552528, -17.65143121711728469, 20.00000000000000000 ) ) ;
#18684=VERTEX_POINT ( 'NONE', #18654 ) ;
#18730=EDGE_CURVE ( 'NONE', #23016, #16381, #2024, .T. ) ;
#18825=DIRECTION ( 'NONE',  ( -1.000000000000000000, 0.000000000000000000, 0.000000000000000000 ) ) ;
#18828=DIRECTION ( 'NONE',  ( 0.000000000000000000, 0.000000000000000000, 1.000000000000000000 ) ) ;
#18845=AXIS2_PLACEMENT_3D ( 'NONE', #10293, #28638, #31305 ) ;
#19072=AXIS2_PLACEMENT_3D ( 'NONE', #22021, #8658, #19536 ) ;
#19138=DIRECTION ( 'NONE',  ( -1.000000000000000000, 0.000000000000000000, 0.000000000000000000 ) ) ;
#19232=CARTESIAN_POINT ( 'NONE',  ( 42.44043929807611448, -17.65143121711728469, 20.00000000000000000 ) ) ;
#19254=ADVANCED_FACE ( 'NONE', ( #8255 ), #30507, .F. ) ;
#19291=EDGE_CURVE ( 'NONE', #30767, #14102, #11833, .T. ) ;
#19293=EDGE_CURVE ( 'NONE', #23708, #34034, #27291, .T. ) ;
#19431=ORIENTED_EDGE ( 'NONE', *, *, #27319, .T. ) ;
#19466=EDGE_LOOP ( 'NONE', ( #21362, #25971 ) ) ;
#19534=DIRECTION ( 'NONE',  ( 0.000000000000000000, 0.000000000000000000, 1.000000000000000000 ) ) ;
#19536=DIRECTION ( 'NONE',  ( 1.000000000000000000, 0.000000000000000000, 0.000000000000000000 ) ) ;
#19540=ORIENTED_EDGE ( 'NONE', *, *, #16552, .F. ) ;
#19555=AXIS2_PLACEMENT_3D ( 'NONE', #19855, #30870, #6476 ) ;
#19569=EDGE_CURVE ( 'NONE', #7759, #23936, #3774, .T. ) ;
#19602=AXIS2_PLACEMENT_3D ( 'NONE', #16206, #24006, #21175 ) ;
#19842=CARTESIAN_POINT ( 'NONE',  ( 28.23027531293552528, -10.15143121711728469, 0.000000000000000000 ) ) ;
#19855=CARTESIAN_POINT ( 'NONE',  ( -35.55956070192387841, -32.65143121711728469, 10.00000000000000000 ) ) ;
#19947=CIRCLE ( 'NONE', #29616, 22.50000000000000355 ) ;
#20054=ORIENTED_EDGE ( 'NONE', *, *, #9535, .T. ) ;
#20062=FACE_OUTER_BOUND ( 'NONE', #27944, .T. ) ;
#20080=CARTESIAN_POINT ( 'NONE',  ( 15.00000000000000000, 1.836970198721029589E-15, 20.00000000000000000 ) ) ;
#20180=CARTESIAN_POINT ( 'NONE',  ( -35.55956070192387841, -17.65143121711728469, 10.00000000000000000 ) ) ;
#20206=CARTESIAN_POINT ( 'NONE',  ( 0.000000000000000000, 0.000000000000000000, 0.000000000000000000 ) ) ;
#20273=DIRECTION ( 'NONE',  ( -0.000000000000000000, -0.000000000000000000, -1.000000000000000000 ) ) ;
#20461=CYLINDRICAL_SURFACE ( 'NONE', #18845, 15.00000000000000000 ) ;
#20701=CARTESIAN_POINT ( 'NONE',  ( -45.05956070192387841, -20.15143121711730245, 20.00000000000000000 ) ) ;
#20727=DIRECTION ( 'NONE',  ( 0.000000000000000000, -0.000000000000000000, -1.000000000000000000 ) ) ;
#20760=VERTEX_POINT ( 'NONE', #9505 ) ;
#20775=EDGE_CURVE ( 'NONE', #15499, #20760, #9841, .T. ) ;
#20869=DIRECTION ( 'NONE',  ( -0.000000000000000000, -0.000000000000000000, -1.000000000000000000 ) ) ;
#20892=CARTESIAN_POINT ( 'NONE',  ( -35.55956070192387841, -17.65143121711728469, 14.30932821646982411 ) ) ;
#20915=DIRECTION ( 'NONE',  ( 1.000000000000000000, 0.000000000000000000, 0.000000000000000000 ) ) ;
#20939=AXIS2_PLACEMENT_3D ( 'NONE', #20701, #1310, #17533 ) ;
#20950=CARTESIAN_POINT ( 'NONE',  ( 35.44043929807611448, -32.65143121711728469, 5.690671783530174999 ) ) ;
#20953=DIRECTION ( 'NONE',  ( 0.000000000000000000, -1.000000000000000000, 0.000000000000000000 ) ) ;
#21030=ORIENTED_EDGE ( 'NONE', *, *, #19293, .F. ) ;
#21175=DIRECTION ( 'NONE',  ( 1.000000000000000000, 0.000000000000000000, 0.000000000000000000 ) ) ;
#21212=DIRECTION ( 'NONE',  ( 0.000000000000000000, 0.000000000000000000, 1.000000000000000000 ) ) ;
#21239=CARTESIAN_POINT ( 'NONE',  ( 0.000000000000000000, 0.000000000000000000, 20.00000000000000000 ) ) ;
#21247=ORIENTED_EDGE ( 'NONE', *, *, #7238, .T. ) ;
#21296=CIRCLE ( 'NONE', #26983, 2.500000000000002220 ) ;
#21362=ORIENTED_EDGE ( 'NONE', *, *, #5624, .T. ) ;
#21392=ORIENTED_EDGE ( 'NONE', *, *, #16096, .T. ) ;
#21398=EDGE_LOOP ( 'NONE', ( #13697, #33656, #26846, #32380 ) ) ;
#21736=ORIENTED_EDGE ( 'NONE', *, *, #22751, .T. ) ;
#21788=LINE ( 'NONE', #11298, #3731 ) ;
#21803=ADVANCED_FACE ( 'NONE', ( #2665 ), #35094, .F. ) ;
#21913=DIRECTION ( 'NONE',  ( -0.000000000000000000, -1.000000000000000000, -0.000000000000000000 ) ) ;
#21952=CIRCLE ( 'NONE', #4884, 4.309328216469825001 ) ;
#22021=CARTESIAN_POINT ( 'NONE',  ( 0.000000000000000000, 0.000000000000000000, 20.00000000000000000 ) ) ;
#22037=ORIENTED_EDGE ( 'NONE', *, *, #32141, .F. ) ;
#22071=CARTESIAN_POINT ( 'NONE',  ( 35.44043929807611448, -32.65143121711728469, 10.00000000000000000 ) ) ;
#22143=CARTESIAN_POINT ( 'NONE',  ( -22.50000000000000355, 0.000000000000000000, 20.00000000000000000 ) ) ;
#22373=DIRECTION ( 'NONE',  ( -1.000000000000000000, 0.000000000000000000, 0.000000000000000000 ) ) ;
#22469=PLANE ( 'NONE',  #6879 ) ;
#22523=CARTESIAN_POINT ( 'NONE',  ( 22.50000000000000355, 2.755455298081545172E-15, 0.000000000000000000 ) ) ;
#22554=ORIENTED_EDGE ( 'NONE', *, *, #29865, .F. ) ;
#22570=LINE ( 'NONE', #8673, #23950 ) ;
#22601=EDGE_LOOP ( 'NONE', ( #5445, #22037 ) ) ;
#22640=ORIENTED_EDGE ( 'NONE', *, *, #16096, .F. ) ;
#22665=ADVANCED_FACE ( 'NONE', ( #11619, #30825 ), #22469, .F. ) ;
#22751=EDGE_CURVE ( 'NONE', #27517, #13700, #8026, .T. ) ;
#22776=DIRECTION ( 'NONE',  ( -0.000000000000000000, -0.000000000000000000, -1.000000000000000000 ) ) ;
#22801=AXIS2_PLACEMENT_3D ( 'NONE', #19842, #30684, #6275 ) ;
#22815=DIRECTION ( 'NONE',  ( -0.000000000000000000, 0.000000000000000000, -1.000000000000000000 ) ) ;
#22831=AXIS2_PLACEMENT_3D ( 'NONE', #4275, #4611, #12491 ) ;
#22867=CARTESIAN_POINT ( 'NONE',  ( -21.17270648470164218, -7.613573412837966181, 0.000000000000000000 ) ) ;
#22968=LINE ( 'NONE', #6926, #30717 ) ;
#23016=VERTEX_POINT ( 'NONE', #1238 ) ;
#23061=APPLICATION_CONTEXT ( 'automotive_design' ) ;
#23100=DIRECTION ( 'NONE',  ( 0.000000000000000000, -0.000000000000000000, -1.000000000000000000 ) ) ;
#23122=CARTESIAN_POINT ( 'NONE',  ( 35.44043929807611448, -32.65143121711728469, 14.30932821646982411 ) ) ;
#23207=AXIS2_PLACEMENT_3D ( 'NONE', #27478, #3267, #14500 ) ;
#23230=AXIS2_PLACEMENT_3D ( 'NONE', #12519, #20869, #33876 ) ;
#23389=PLANE ( 'NONE',  #32464 ) ;
#23405=AXIS2_PLACEMENT_3D ( 'NONE', #12252, #26449, #23100 ) ;
#23419=ADVANCED_FACE ( 'NONE', ( #1884, #4017 ), #12248, .T. ) ;
#23458=LINE ( 'NONE', #25469, #2056 ) ;
#23467=ADVANCED_FACE ( 'NONE', ( #29302 ), #5591, .F. ) ;
#23490=ORIENTED_EDGE ( 'NONE', *, *, #17476, .F. ) ;
#23542=CARTESIAN_POINT ( 'NONE',  ( 44.94043929807611448, -32.65143121711728469, 0.000000000000000000 ) ) ;
#23543=CARTESIAN_POINT ( 'NONE',  ( -35.55956070192387841, -12.65143121711728291, 14.30932821646982411 ) ) ;
#23708=VERTEX_POINT ( 'NONE', #17846 ) ;
#23841=DIRECTION ( 'NONE',  ( -0.000000000000000000, -0.000000000000000000, -1.000000000000000000 ) ) ;
#23936=VERTEX_POINT ( 'NONE', #1417 ) ;
#23948=CIRCLE ( 'NONE', #24524, 2.500000000000002220 ) ;
#23950=VECTOR ( 'NONE', #1196, 1000.000000000000000 ) ;
#23974=DIRECTION ( 'NONE',  ( 0.000000000000000000, 0.000000000000000000, -1.000000000000000000 ) ) ;
#23997=CARTESIAN_POINT ( 'NONE',  ( -35.55956070192387841, -12.65143121711728291, 10.00000000000000000 ) ) ;
#24006=DIRECTION ( 'NONE',  ( 0.000000000000000000, 0.000000000000000000, 1.000000000000000000 ) ) ;
#24100=ADVANCED_FACE ( 'NONE', ( #4576 ), #20461, .F. ) ;
#24131=DIRECTION ( 'NONE',  ( -0.000000000000000000, -0.000000000000000000, -1.000000000000000000 ) ) ;
#24146=EDGE_CURVE ( 'NONE', #1315, #34034, #29063, .T. ) ;
#24176=VECTOR ( 'NONE', #26776, 1000.000000000000000 ) ;
#24371=EDGE_CURVE ( 'NONE', #34682, #25632, #22570, .T. ) ;
#24418=ORIENTED_EDGE ( 'NONE', *, *, #29080, .T. ) ;
#24452=CIRCLE ( 'NONE', #29013, 4.309328216469825001 ) ;
#24473=DIRECTION ( 'NONE',  ( -0.000000000000000000, -0.000000000000000000, -1.000000000000000000 ) ) ;
#24508=EDGE_LOOP ( 'NONE', ( #6422, #19540, #11690, #17572 ) ) ;
#24524=AXIS2_PLACEMENT_3D ( 'NONE', #25776, #1579, #3536 ) ;
#24542=LINE ( 'NONE', #30434, #29440 ) ;
#24547=DIRECTION ( 'NONE',  ( -0.000000000000000000, -0.000000000000000000, -1.000000000000000000 ) ) ;
#24559=ADVANCED_FACE ( 'NONE', ( #1887, #12768 ), #15612, .F. ) ;
#24642=ADVANCED_FACE ( 'NONE', ( #29306 ), #98, .F. ) ;
#24645=ADVANCED_FACE ( 'NONE', ( #13457 ), #5074, .F. ) ;
#24674=ORIENTED_EDGE ( 'NONE', *, *, #33065, .F. ) ;
#24708=CIRCLE ( 'NONE', #19602, 15.00000000000000000 ) ;
#24911=VECTOR ( 'NONE', #16428, 1000.000000000000000 ) ;
#24918=CARTESIAN_POINT ( 'NONE',  ( -35.55956070192387841, -12.65143121711728291, 5.690671783530174999 ) ) ;
#24981=DIRECTION ( 'NONE',  ( 0.000000000000000000, 0.000000000000000000, 1.000000000000000000 ) ) ;
#24989=ORIENTED_EDGE ( 'NONE', *, *, #14612, .F. ) ;
#25040=AXIS2_PLACEMENT_3D ( 'NONE', #29997, #26445, #32307 ) ;
#25070=AXIS2_PLACEMENT_3D ( 'NONE', #4161, #15050, #7177 ) ;
#25119=DIRECTION ( 'NONE',  ( 1.000000000000000000, 0.000000000000000000, 0.000000000000000000 ) ) ;
#25200=VECTOR ( 'NONE', #12846, 1000.000000000000000 ) ;
#25231=ORIENTED_EDGE ( 'NONE', *, *, #32141, .T. ) ;
#25273=VERTEX_POINT ( 'NONE', #5064 ) ;
#25347=ORIENTED_EDGE ( 'NONE', *, *, #2512, .F. ) ;
#25440=CARTESIAN_POINT ( 'NONE',  ( 21.17270648470164218, -7.613573412837960852, 20.00000000000000000 ) ) ;
#25469=CARTESIAN_POINT ( 'NONE',  ( 44.94043929807611448, -32.65143121711728469, 20.00000000000000000 ) ) ;
#25616=ORIENTED_EDGE ( 'NONE', *, *, #12403, .F. ) ;
#25632=VERTEX_POINT ( 'NONE', #10202 ) ;
#25733=DIRECTION ( 'NONE',  ( 0.000000000000000000, -0.000000000000000000, 1.000000000000000000 ) ) ;
#25776=CARTESIAN_POINT ( 'NONE',  ( -42.55956070192387841, -20.15143121711728469, 20.00000000000000000 ) ) ;
#25862=FACE_OUTER_BOUND ( 'NONE', #18422, .T. ) ;
#25971=ORIENTED_EDGE ( 'NONE', *, *, #15080, .T. ) ;
#25980=VERTEX_POINT ( 'NONE', #7470 ) ;
#26043=EDGE_CURVE ( 'NONE', #1246, #17344, #6779, .T. ) ;
#26062=CYLINDRICAL_SURFACE ( 'NONE', #25070, 22.50000000000000355 ) ;
#26360=CIRCLE ( 'NONE', #32606, 15.00000000000000000 ) ;
#26404=ORIENTED_EDGE ( 'NONE', *, *, #33790, .F. ) ;
#26426=VERTEX_POINT ( 'NONE', #15127 ) ;
#26445=DIRECTION ( 'NONE',  ( -0.000000000000000000, -1.000000000000000000, -0.000000000000000000 ) ) ;
#26449=DIRECTION ( 'NONE',  ( 0.000000000000000000, -1.000000000000000000, 0.000000000000000000 ) ) ;
#26455=ORIENTED_EDGE ( 'NONE', *, *, #19569, .T. ) ;
#26508=AXIS2_PLACEMENT_3D ( 'NONE', #10012, #31716, #13219 ) ;
#26559=LINE ( 'NONE', #10195, #34749 ) ;
#26579=CARTESIAN_POINT ( 'NONE',  ( 0.000000000000000000, 0.000000000000000000, 0.000000000000000000 ) ) ;
#26623=DIRECTION ( 'NONE',  ( -0.000000000000000000, -1.000000000000000000, -0.000000000000000000 ) ) ;
#26627=CIRCLE ( 'NONE', #6732, 2.500000000000002220 ) ;
#26632=ORIENTED_EDGE ( 'NONE', *, *, #12799, .F. ) ;
#26680=FACE_OUTER_BOUND ( 'NONE', #29224, .T. ) ;
#26730=CARTESIAN_POINT ( 'NONE',  ( 44.94043929807611448, -20.15143121711728469, 20.00000000000000000 ) ) ;
#26776=DIRECTION ( 'NONE',  ( -1.000000000000000000, -0.000000000000000000, -0.000000000000000000 ) ) ;
#26821=CIRCLE ( 'NONE', #14349, 2.500000000000002220 ) ;
#26846=ORIENTED_EDGE ( 'NONE', *, *, #30777, .T. ) ;
#26852=CIRCLE ( 'NONE', #13250, 4.309328216469825001 ) ;
#26983=AXIS2_PLACEMENT_3D ( 'NONE', #27452, #754, #25119 ) ;
#27013=VECTOR ( 'NONE', #7968, 1000.000000000000000 ) ;
#27068=ORIENTED_EDGE ( 'NONE', *, *, #30006, .F. ) ;
#27219=ORIENTED_EDGE ( 'NONE', *, *, #24146, .T. ) ;
#27223=AXIS2_PLACEMENT_3D ( 'NONE', #18569, #21212, #28400 ) ;
#27273=ADVANCED_FACE ( 'NONE', ( #31349 ), #6956, .F. ) ;
#27291=LINE ( 'NONE', #22143, #3190 ) ;
#27319=EDGE_CURVE ( 'NONE', #27517, #16381, #16753, .T. ) ;
#27452=CARTESIAN_POINT ( 'NONE',  ( -42.55956070192387841, -20.15143121711728469, 0.000000000000000000 ) ) ;
#27478=CARTESIAN_POINT ( 'NONE',  ( 0.000000000000000000, 0.000000000000000000, 20.00000000000000000 ) ) ;
#27510=DIRECTION ( 'NONE',  ( -0.000000000000000000, -0.000000000000000000, -1.000000000000000000 ) ) ;
#27517=VERTEX_POINT ( 'NONE', #25440 ) ;
#27527=DIRECTION ( 'NONE',  ( 1.000000000000000000, 0.000000000000000000, 0.000000000000000000 ) ) ;
#27581=DIRECTION ( 'NONE',  ( -0.000000000000000000, -0.000000000000000000, -1.000000000000000000 ) ) ;
#27595=ORIENTED_EDGE ( 'NONE', *, *, #3726, .F. ) ;
#27609=AXIS2_PLACEMENT_3D ( 'NONE', #9842, #7509, #29240 ) ;
#27653=CYLINDRICAL_SURFACE ( 'NONE', #23207, 22.50000000000000355 ) ;
#27742=ORIENTED_EDGE ( 'NONE', *, *, #15404, .T. ) ;
#27774=LINE ( 'NONE', #24918, #13093 ) ;
#27793=ORIENTED_EDGE ( 'NONE', *, *, #7238, .F. ) ;
#27807=EDGE_CURVE ( 'NONE', #13700, #1315, #34870, .T. ) ;
#27825=DIRECTION ( 'NONE',  ( -0.000000000000000000, -0.000000000000000000, -1.000000000000000000 ) ) ;
#27875=CARTESIAN_POINT ( 'NONE',  ( 0.000000000000000000, 0.000000000000000000, 20.00000000000000000 ) ) ;
#27908=VERTEX_POINT ( 'NONE', #20080 ) ;
#27933=CARTESIAN_POINT ( 'NONE',  ( -42.55956070192386420, -17.65143121711728469, 20.00000000000000000 ) ) ;
#27944=EDGE_LOOP ( 'NONE', ( #28965, #23490, #25616, #30949 ) ) ;
#27972=CARTESIAN_POINT ( 'NONE',  ( -45.05956070192387841, -20.15143121711730245, 20.00000000000000000 ) ) ;
#28004=DIRECTION ( 'NONE',  ( -0.000000000000000000, -0.000000000000000000, -1.000000000000000000 ) ) ;
#28066=EDGE_LOOP ( 'NONE', ( #25347, #9779, #7134, #3005 ) ) ;
#28211=FACE_OUTER_BOUND ( 'NONE', #17339, .T. ) ;
#28261=AXIS2_PLACEMENT_3D ( 'NONE', #34479, #20953, #31797 ) ;
#28263=ORIENTED_EDGE ( 'NONE', *, *, #24146, .F. ) ;
#28275=ADVANCED_FACE ( 'NONE', ( #7751 ), #29481, .T. ) ;
#28276=CARTESIAN_POINT ( 'NONE',  ( 44.94043929807611448, -32.65143121711728469, 0.000000000000000000 ) ) ;
#28313=CARTESIAN_POINT ( 'NONE',  ( -15.00000000000000000, 0.000000000000000000, 0.000000000000000000 ) ) ;
#28400=DIRECTION ( 'NONE',  ( 1.000000000000000000, 0.000000000000000000, 0.000000000000000000 ) ) ;
#28468=UNCERTAINTY_MEASURE_WITH_UNIT (LENGTH_MEASURE( 1.000000000000000082E-05 ), #14663, 'distance_accuracy_value', 'NONE');
#28472=ADVANCED_FACE ( 'NONE', ( #13205 ), #26062, .T. ) ;
#28522=ADVANCED_FACE ( 'NONE', ( #32233, #28211 ), #23389, .F. ) ;
#28527=ORIENTED_EDGE ( 'NONE', *, *, #15800, .T. ) ;
#28566=AXIS2_PLACEMENT_3D ( 'NONE', #26579, #2200, #13073 ) ;
#28638=DIRECTION ( 'NONE',  ( -0.000000000000000000, -0.000000000000000000, -1.000000000000000000 ) ) ;
#28659=EDGE_CURVE ( 'NONE', #17344, #15610, #24452, .T. ) ;
#28681=DIRECTION ( 'NONE',  ( -1.000000000000000000, 0.000000000000000000, 0.000000000000000000 ) ) ;
#28755=PLANE ( 'NONE',  #17383 ) ;
#28893=DIRECTION ( 'NONE',  ( 1.000000000000000000, 0.000000000000000000, 0.000000000000000000 ) ) ;
#28928=ORIENTED_EDGE ( 'NONE', *, *, #33065, .T. ) ;
#28929=MECHANICAL_DESIGN_GEOMETRIC_PRESENTATION_REPRESENTATION('',(#9037),#11332);
#28965=ORIENTED_EDGE ( 'NONE', *, *, #13144, .T. ) ;
#29013=AXIS2_PLACEMENT_3D ( 'NONE', #16413, #193, #11232 ) ;
#29063=CIRCLE ( 'NONE', #673, 22.50000000000000355 ) ;
#29071=ORIENTED_EDGE ( 'NONE', *, *, #27807, .F. ) ;
#29080=EDGE_CURVE ( 'NONE', #7524, #23016, #29607, .T. ) ;
#29121=AXIS2_PLACEMENT_3D ( 'NONE', #35004, #4899, #5426 ) ;
#29139=CARTESIAN_POINT ( 'NONE',  ( 0.000000000000000000, 0.000000000000000000, 20.00000000000000000 ) ) ;
#29221=LINE ( 'NONE', #13212, #11955 ) ;
#29224=EDGE_LOOP ( 'NONE', ( #33800, #15258, #25231, #588 ) ) ;
#29240=DIRECTION ( 'NONE',  ( -1.000000000000000000, 0.000000000000000000, 0.000000000000000000 ) ) ;
#29302=FACE_OUTER_BOUND ( 'NONE', #14946, .T. ) ;
#29306=FACE_OUTER_BOUND ( 'NONE', #10581, .T. ) ;
#29317=CARTESIAN_POINT ( 'NONE',  ( -35.55956070192387841, -17.65143121711728469, 5.690671783530174999 ) ) ;
#29342=EDGE_CURVE ( 'NONE', #15960, #15610, #34753, .T. ) ;
#29408=ORIENTED_EDGE ( 'NONE', *, *, #30005, .T. ) ;
#29440=VECTOR ( 'NONE', #27581, 1000.000000000000000 ) ;
#29481=CYLINDRICAL_SURFACE ( 'NONE', #2360, 2.500000000000002220 ) ;
#29590=FACE_OUTER_BOUND ( 'NONE', #10358, .T. ) ;
#29607=CIRCLE ( 'NONE', #22801, 7.500000000000000000 ) ;
#29616=AXIS2_PLACEMENT_3D ( 'NONE', #34267, #12564, #20915 ) ;
#29865=EDGE_CURVE ( 'NONE', #32903, #11385, #33015, .T. ) ;
#29869=CLOSED_SHELL ( 'NONE', ( #2158, #24645, #11330, #11980, #34063, #24642, #22665, #23419, #12058, #28472, #19254, #24559, #7443, #12034, #6904, #27273, #28275, #28522, #24100, #23467, #21803 ) ) ;
#29888=VERTEX_POINT ( 'NONE', #19232 ) ;
#29902=DIRECTION ( 'NONE',  ( -0.000000000000000000, -0.000000000000000000, -1.000000000000000000 ) ) ;
#29997=CARTESIAN_POINT ( 'NONE',  ( 35.44043929807611448, -12.65143121711728291, 10.00000000000000000 ) ) ;
#30005=EDGE_CURVE ( 'NONE', #33194, #26426, #23948, .T. ) ;
#30006=EDGE_CURVE ( 'NONE', #18684, #33194, #7075, .T. ) ;
#30070=ORIENTED_EDGE ( 'NONE', *, *, #18730, .F. ) ;
#30241=DIRECTION ( 'NONE',  ( -1.000000000000000000, 0.000000000000000000, 0.000000000000000000 ) ) ;
#30246=EDGE_CURVE ( 'NONE', #25980, #9992, #4073, .T. ) ;
#30316=DIRECTION ( 'NONE',  ( 0.000000000000000000, 0.000000000000000000, -1.000000000000000000 ) ) ;
#30332=PRODUCT_DEFINITION ( 'UNKNOWN', '', #9884, #34916 ) ;
#30434=CARTESIAN_POINT ( 'NONE',  ( 28.23027531293552528, -17.65143121711728469, 20.00000000000000000 ) ) ;
#30490=( NAMED_UNIT ( * ) PLANE_ANGLE_UNIT ( ) SI_UNIT ( $, .RADIAN. ) );
#30507=CYLINDRICAL_SURFACE ( 'NONE', #34447, 7.500000000000000000 ) ;
#30551=ORIENTED_EDGE ( 'NONE', *, *, #12907, .T. ) ;
#30665=ORIENTED_EDGE ( 'NONE', *, *, #16552, .T. ) ;
#30684=DIRECTION ( 'NONE',  ( -0.000000000000000000, -0.000000000000000000, -1.000000000000000000 ) ) ;
#30693=CARTESIAN_POINT ( 'NONE',  ( 0.000000000000000000, 0.000000000000000000, 0.000000000000000000 ) ) ;
#30717=VECTOR ( 'NONE', #33993, 1000.000000000000000 ) ;
#30767=VERTEX_POINT ( 'NONE', #14862 ) ;
#30777=EDGE_CURVE ( 'NONE', #34034, #32903, #33667, .T. ) ;
#30825=FACE_BOUND ( 'NONE', #4893, .T. ) ;
#30838=SHAPE_REPRESENTATION_RELATIONSHIP ( 'NONE' , 'NONE' ,  #11185, #32214 ) ;
#30857=CARTESIAN_POINT ( 'NONE',  ( 21.17270648470164218, -7.613573412837960852, 0.000000000000000000 ) ) ;
#30870=DIRECTION ( 'NONE',  ( 0.000000000000000000, -1.000000000000000000, 0.000000000000000000 ) ) ;
#30938=ORIENTED_EDGE ( 'NONE', *, *, #35041, .F. ) ;
#30948=LINE ( 'NONE', #9421, #24911 ) ;
#30949=ORIENTED_EDGE ( 'NONE', *, *, #3726, .T. ) ;
#31015=( NAMED_UNIT ( * ) SI_UNIT ( $, .STERADIAN. ) SOLID_ANGLE_UNIT ( ) );
#31070=EDGE_CURVE ( 'NONE', #15610, #17344, #26852, .T. ) ;
#31134=AXIS2_PLACEMENT_3D ( 'NONE', #29139, #34664, #10271 ) ;
#31250=CARTESIAN_POINT ( 'NONE',  ( 35.44043929807611448, -17.65143121711728469, 14.30932821646982411 ) ) ;
#31305=DIRECTION ( 'NONE',  ( -1.000000000000000000, 0.000000000000000000, 0.000000000000000000 ) ) ;
#31349=FACE_OUTER_BOUND ( 'NONE', #5355, .T. ) ;
#31447=VERTEX_POINT ( 'NONE', #4572 ) ;
#31479=AXIS2_PLACEMENT_3D ( 'NONE', #20206, #6823, #28893 ) ;
#31623=CIRCLE ( 'NONE', #19072, 22.50000000000000355 ) ;
#31637=ORIENTED_EDGE ( 'NONE', *, *, #13818, .F. ) ;
#31683=CARTESIAN_POINT ( 'NONE',  ( 35.44043929807611448, -12.65143121711728291, 5.690671783530174999 ) ) ;
#31716=DIRECTION ( 'NONE',  ( 0.000000000000000000, -1.000000000000000000, 0.000000000000000000 ) ) ;
#31724=CARTESIAN_POINT ( 'NONE',  ( 28.23027531293552528, -17.65143121711728469, 0.000000000000000000 ) ) ;
#31734=ORIENTED_EDGE ( 'NONE', *, *, #20775, .F. ) ;
#31797=DIRECTION ( 'NONE',  ( 0.000000000000000000, 0.000000000000000000, -1.000000000000000000 ) ) ;
#31879=ORIENTED_EDGE ( 'NONE', *, *, #9038, .T. ) ;
#31903=ORIENTED_EDGE ( 'NONE', *, *, #24371, .T. ) ;
#31933=UNCERTAINTY_MEASURE_WITH_UNIT (LENGTH_MEASURE( 1.000000000000000082E-05 ), #8204, 'distance_accuracy_value', 'NONE');
#32052=DIRECTION ( 'NONE',  ( -0.000000000000000000, -0.000000000000000000, -1.000000000000000000 ) ) ;
#32062=CARTESIAN_POINT ( 'NONE',  ( 28.23027531293552528, -17.65143121711728469, 0.000000000000000000 ) ) ;
#32067=CARTESIAN_POINT ( 'NONE',  ( 15.00000000000000000, 1.836970198721029589E-15, 0.000000000000000000 ) ) ;
#32141=EDGE_CURVE ( 'NONE', #23936, #7759, #15563, .T. ) ;
#32161=VECTOR ( 'NONE', #5186, 1000.000000000000000 ) ;
#32214=ADVANCED_BREP_SHAPE_REPRESENTATION ( '', ( #10712, #28566 ), #10929 ) ;
#32233=FACE_BOUND ( 'NONE', #15868, .T. ) ;
#32248=CARTESIAN_POINT ( 'NONE',  ( 35.44043929807611448, -12.65143121711728291, 14.30932821646982411 ) ) ;
#32307=DIRECTION ( 'NONE',  ( 0.000000000000000000, 0.000000000000000000, -1.000000000000000000 ) ) ;
#32352=DIRECTION ( 'NONE',  ( 0.000000000000000000, 0.000000000000000000, 1.000000000000000000 ) ) ;
#32380=ORIENTED_EDGE ( 'NONE', *, *, #12907, .F. ) ;
#32464=AXIS2_PLACEMENT_3D ( 'NONE', #34247, #9862, #20727 ) ;
#32492=LINE ( 'NONE', #7760, #32626 ) ;
#32579=PRODUCT_CONTEXT ( 'NONE', #23061, 'mechanical' ) ;
#32606=AXIS2_PLACEMENT_3D ( 'NONE', #335, #10669, #14036 ) ;
#32626=VECTOR ( 'NONE', #24131, 1000.000000000000000 ) ;
#32637=DIRECTION ( 'NONE',  ( -1.000000000000000000, -0.000000000000000000, -0.000000000000000000 ) ) ;
#32770=EDGE_CURVE ( 'NONE', #4571, #14102, #2505, .T. ) ;
#32889=AXIS2_PLACEMENT_3D ( 'NONE', #27875, #19534, #27527 ) ;
#32903=VERTEX_POINT ( 'NONE', #22867 ) ;
#32913=ORIENTED_EDGE ( 'NONE', *, *, #31070, .F. ) ;
#32945=EDGE_LOOP ( 'NONE', ( #7048, #10085, #2374, #26455 ) ) ;
#32974=ORIENTED_EDGE ( 'NONE', *, *, #7854, .F. ) ;
#33015=CIRCLE ( 'NONE', #5746, 7.500000000000000000 ) ;
#33065=EDGE_CURVE ( 'NONE', #31447, #34682, #21296, .T. ) ;
#33189=CARTESIAN_POINT ( 'NONE',  ( 35.44043929807611448, -17.65143121711728469, 5.690671783530174999 ) ) ;
#33194=VERTEX_POINT ( 'NONE', #4099 ) ;
#33386=ORIENTED_EDGE ( 'NONE', *, *, #14026, .F. ) ;
#33395=AXIS2_PLACEMENT_3D ( 'NONE', #15068, #7022, #17575 ) ;
#33412=DIRECTION ( 'NONE',  ( -0.000000000000000000, -0.000000000000000000, -1.000000000000000000 ) ) ;
#33467=ORIENTED_EDGE ( 'NONE', *, *, #9038, .F. ) ;
#33529=DIRECTION ( 'NONE',  ( -0.000000000000000000, -0.000000000000000000, -1.000000000000000000 ) ) ;
#33538=CARTESIAN_POINT ( 'NONE',  ( -45.05956070192387841, -20.15143121711730245, 20.00000000000000000 ) ) ;
#33656=ORIENTED_EDGE ( 'NONE', *, *, #19293, .T. ) ;
#33661=DIRECTION ( 'NONE',  ( 0.000000000000000000, -1.000000000000000000, 0.000000000000000000 ) ) ;
#33667=CIRCLE ( 'NONE', #11495, 22.50000000000000355 ) ;
#33695=PLANE ( 'NONE',  #20939 ) ;
#33790=EDGE_CURVE ( 'NONE', #26426, #34682, #11140, .T. ) ;
#33800=ORIENTED_EDGE ( 'NONE', *, *, #15080, .F. ) ;
#33876=DIRECTION ( 'NONE',  ( -1.000000000000000000, 0.000000000000000000, 0.000000000000000000 ) ) ;
#33993=DIRECTION ( 'NONE',  ( -0.000000000000000000, -0.000000000000000000, -1.000000000000000000 ) ) ;
#34001=EDGE_LOOP ( 'NONE', ( #2062, #7601 ) ) ;
#34034=VERTEX_POINT ( 'NONE', #18238 ) ;
#34063=ADVANCED_FACE ( 'NONE', ( #7706 ), #9855, .T. ) ;
#34128=CARTESIAN_POINT ( 'NONE',  ( 28.23027531293552528, -10.15143121711728469, 20.00000000000000000 ) ) ;
#34225=ORIENTED_EDGE ( 'NONE', *, *, #29342, .F. ) ;
#34247=CARTESIAN_POINT ( 'NONE',  ( 28.23027531293552528, -17.65143121711728469, 20.00000000000000000 ) ) ;
#34267=CARTESIAN_POINT ( 'NONE',  ( 0.000000000000000000, 0.000000000000000000, 20.00000000000000000 ) ) ;
#34272=DIRECTION ( 'NONE',  ( -0.000000000000000000, -0.000000000000000000, -1.000000000000000000 ) ) ;
#34354=EDGE_LOOP ( 'NONE', ( #15244, #17072, #13851, #31734, #15272, #10261, #24674, #5995, #22554, #17418, #28263, #17819, #30070 ) ) ;
#34447=AXIS2_PLACEMENT_3D ( 'NONE', #17172, #27825, #19138 ) ;
#34479=CARTESIAN_POINT ( 'NONE',  ( 35.44043929807611448, -17.65143121711728469, 10.00000000000000000 ) ) ;
#34664=DIRECTION ( 'NONE',  ( -0.000000000000000000, -0.000000000000000000, -1.000000000000000000 ) ) ;
#34682=VERTEX_POINT ( 'NONE', #9610 ) ;
#34690=VERTEX_POINT ( 'NONE', #1590 ) ;
#34745=DIRECTION ( 'NONE',  ( -1.000000000000000000, -0.000000000000000000, -0.000000000000000000 ) ) ;
#34749=VECTOR ( 'NONE', #13052, 1000.000000000000000 ) ;
#34753=LINE ( 'NONE', #32248, #14833 ) ;
#34870=LINE ( 'NONE', #18512, #27013 ) ;
#34916=PRODUCT_DEFINITION_CONTEXT ( 'detailed design', #15794, 'design' ) ;
#35004=CARTESIAN_POINT ( 'NONE',  ( 28.23027531293552528, -10.15143121711728469, 20.00000000000000000 ) ) ;
#35041=EDGE_CURVE ( 'NONE', #12488, #18684, #720, .T. ) ;
#35054=ORIENTED_EDGE ( 'NONE', *, *, #6166, .T. ) ;
#35094=CYLINDRICAL_SURFACE ( 'NONE', #987, 4.309328216469825001 ) ;
#35269=COLOUR_RGB('Grey',0.48,0.52,0.57);
#35270=FILL_AREA_STYLE_COLOUR('',#35269);
#35271=FILL_AREA_STYLE('',(#35270));
#35272=SURFACE_STYLE_FILL_AREA(#35271);
#35273=SURFACE_SIDE_STYLE('',(#35272));
#35274=SURFACE_STYLE_USAGE(.BOTH.,#35273);
#35275=PRESENTATION_STYLE_ASSIGNMENT((#35274));
ENDSEC;
END-ISO-10303-21;
